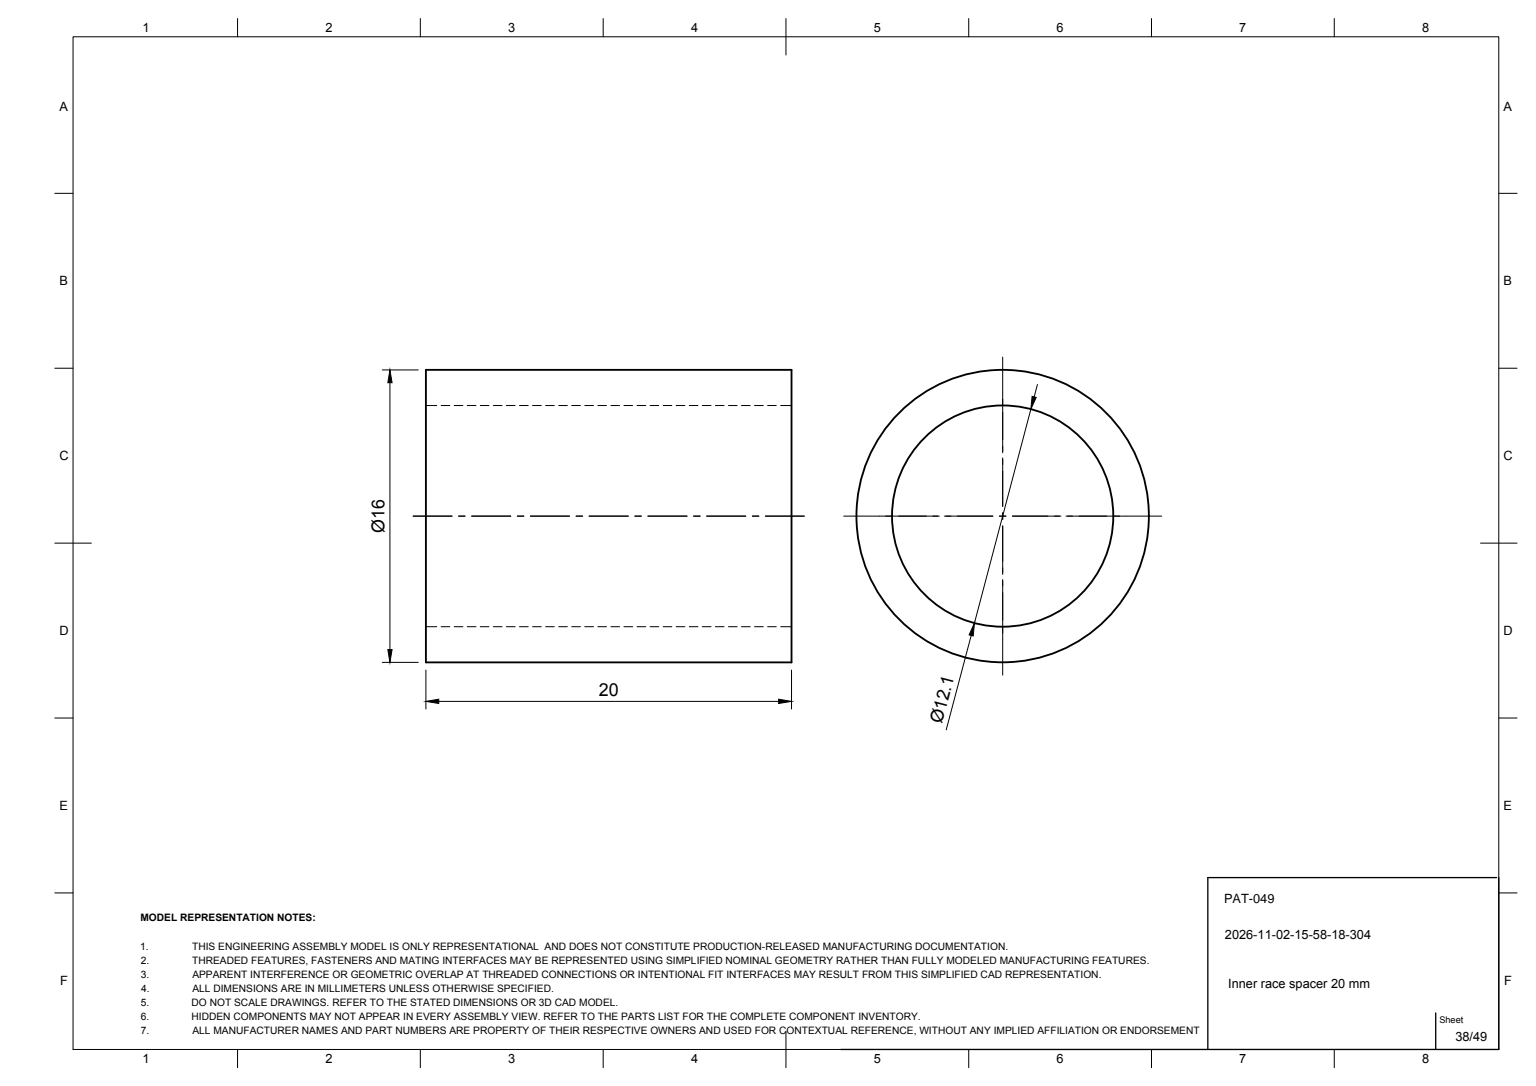
ISO-10303-21;
HEADER;
/* Generated by software containing ST-Developer
 * from STEP Tools, Inc. (www.steptools.com) 
 */

FILE_DESCRIPTION(
/* description */ ('Hand drill press frame (manual)'),
/* implementation_level */ '2;1');

FILE_NAME(
/* name */ 'Inner race spacer 20 mm.step',
/* time_stamp */ '2026-10-28T03:25:28-07:00',
/* author */ (''),
/* organization */ (''),
/* preprocessor_version */ 'ST-DEVELOPER v20.2',
/* originating_system */ 'Autodesk Translation Framework v15.17.0.0',
/* authorisation */ '');

FILE_SCHEMA (('AUTOMOTIVE_DESIGN { 1 0 10303 214 3 1 1 }'));
ENDSEC;

DATA;
#10=MECHANICAL_DESIGN_GEOMETRIC_PRESENTATION_REPRESENTATION('',(#656),#33299);
#559=SHAPE_REPRESENTATION_RELATIONSHIP('SRR','None',#33521,#604);
#604=ADVANCED_BREP_SHAPE_REPRESENTATION('',(#707),#33283);
#656=STYLED_ITEM('',(#33814),#707);
#707=MANIFOLD_SOLID_BREP('Body1',#12675);
#859=FACE_BOUND('',#2676,.T.);
#860=FACE_BOUND('',#2678,.T.);
#1252=PLANE('',#14040);
#1253=PLANE('',#14041);
#1845=FACE_OUTER_BOUND('',#2673,.T.);
#1846=FACE_OUTER_BOUND('',#2674,.T.);
#1847=FACE_OUTER_BOUND('',#2675,.T.);
#1848=FACE_OUTER_BOUND('',#2677,.T.);
#2673=EDGE_LOOP('',(#10931,#10932,#10933,#10934));
#2674=EDGE_LOOP('',(#10935,#10936,#10937,#10938));
#2675=EDGE_LOOP('',(#10939));
#2676=EDGE_LOOP('',(#10940));
#2677=EDGE_LOOP('',(#10941));
#2678=EDGE_LOOP('',(#10942));
#3808=LINE('',#21144,#4973);
#3809=LINE('',#21150,#4974);
#4973=VECTOR('',#16987,0.605);
#4974=VECTOR('',#16994,0.8);
#5507=CIRCLE('',#14035,0.605);
#5508=CIRCLE('',#14036,0.605);
#5509=CIRCLE('',#14038,0.8);
#5510=CIRCLE('',#14039,0.8);
#6457=VERTEX_POINT('',#21141);
#6458=VERTEX_POINT('',#21143);
#6459=VERTEX_POINT('',#21147);
#6460=VERTEX_POINT('',#21149);
#7994=EDGE_CURVE('',#6457,#6457,#5507,.T.);
#7995=EDGE_CURVE('',#6457,#6458,#3808,.T.);
#7996=EDGE_CURVE('',#6458,#6458,#5508,.T.);
#7997=EDGE_CURVE('',#6459,#6459,#5509,.T.);
#7998=EDGE_CURVE('',#6459,#6460,#3809,.T.);
#7999=EDGE_CURVE('',#6460,#6460,#5510,.T.);
#10931=ORIENTED_EDGE('',*,*,#7994,.F.);
#10932=ORIENTED_EDGE('',*,*,#7995,.T.);
#10933=ORIENTED_EDGE('',*,*,#7996,.T.);
#10934=ORIENTED_EDGE('',*,*,#7995,.F.);
#10935=ORIENTED_EDGE('',*,*,#7997,.F.);
#10936=ORIENTED_EDGE('',*,*,#7998,.T.);
#10937=ORIENTED_EDGE('',*,*,#7999,.T.);
#10938=ORIENTED_EDGE('',*,*,#7998,.F.);
#10939=ORIENTED_EDGE('',*,*,#7997,.T.);
#10940=ORIENTED_EDGE('',*,*,#7994,.T.);
#10941=ORIENTED_EDGE('',*,*,#7999,.F.);
#10942=ORIENTED_EDGE('',*,*,#7996,.F.);
#11900=CYLINDRICAL_SURFACE('',#14034,0.605);
#11901=CYLINDRICAL_SURFACE('',#14037,0.8);
#12454=ADVANCED_FACE('',(#1845),#11900,.F.);
#12455=ADVANCED_FACE('',(#1846),#11901,.T.);
#12456=ADVANCED_FACE('',(#1847,#859),#1252,.T.);
#12457=ADVANCED_FACE('',(#1848,#860),#1253,.F.);
#12675=CLOSED_SHELL('',(#12454,#12455,#12456,#12457));
#14033=AXIS2_PLACEMENT_3D('',#21139,#16981,#16982);
#14034=AXIS2_PLACEMENT_3D('',#21140,#16983,#16984);
#14035=AXIS2_PLACEMENT_3D('',#21142,#16985,#16986);
#14036=AXIS2_PLACEMENT_3D('',#21145,#16988,#16989);
#14037=AXIS2_PLACEMENT_3D('',#21146,#16990,#16991);
#14038=AXIS2_PLACEMENT_3D('',#21148,#16992,#16993);
#14039=AXIS2_PLACEMENT_3D('',#21151,#16995,#16996);
#14040=AXIS2_PLACEMENT_3D('',#21152,#16997,#16998);
#14041=AXIS2_PLACEMENT_3D('',#21153,#16999,#17000);
#16981=DIRECTION('axis',(0.,0.,1.));
#16982=DIRECTION('refdir',(1.,0.,0.));
#16983=DIRECTION('center_axis',(0.,1.,0.));
#16984=DIRECTION('ref_axis',(1.,0.,0.));
#16985=DIRECTION('center_axis',(0.,-1.,0.));
#16986=DIRECTION('ref_axis',(1.,0.,0.));
#16987=DIRECTION('',(0.,-1.,0.));
#16988=DIRECTION('center_axis',(0.,-1.,0.));
#16989=DIRECTION('ref_axis',(1.,0.,0.));
#16990=DIRECTION('center_axis',(0.,1.,0.));
#16991=DIRECTION('ref_axis',(1.,0.,0.));
#16992=DIRECTION('center_axis',(0.,1.,0.));
#16993=DIRECTION('ref_axis',(1.,0.,0.));
#16994=DIRECTION('',(0.,-1.,0.));
#16995=DIRECTION('center_axis',(0.,1.,0.));
#16996=DIRECTION('ref_axis',(1.,0.,0.));
#16997=DIRECTION('center_axis',(0.,1.,0.));
#16998=DIRECTION('ref_axis',(1.,0.,0.));
#16999=DIRECTION('center_axis',(0.,1.,0.));
#17000=DIRECTION('ref_axis',(1.,0.,0.));
#21139=CARTESIAN_POINT('',(0.,0.,0.));
#21140=CARTESIAN_POINT('Origin',(-3.25,-5.5,20.));
#21141=CARTESIAN_POINT('',(-3.855,-3.5,20.));
#21142=CARTESIAN_POINT('Origin',(-3.25,-3.5,20.));
#21143=CARTESIAN_POINT('',(-3.855,-5.5,20.));
#21144=CARTESIAN_POINT('',(-3.855,-5.5,20.));
#21145=CARTESIAN_POINT('Origin',(-3.25,-5.5,20.));
#21146=CARTESIAN_POINT('Origin',(-3.25,-5.5,20.));
#21147=CARTESIAN_POINT('',(-4.05,-3.5,20.));
#21148=CARTESIAN_POINT('Origin',(-3.25,-3.5,20.));
#21149=CARTESIAN_POINT('',(-4.05,-5.5,20.));
#21150=CARTESIAN_POINT('',(-4.05,-5.5,20.));
#21151=CARTESIAN_POINT('Origin',(-3.25,-5.5,20.));
#21152=CARTESIAN_POINT('Origin',(-3.25,-3.5,20.));
#21153=CARTESIAN_POINT('Origin',(-3.25,-5.5,20.));
#33231=UNCERTAINTY_MEASURE_WITH_UNIT(LENGTH_MEASURE(0.001),#33300,
'DISTANCE_ACCURACY_VALUE',
'Maximum model space distance between geometric entities at asserted c
onnectivities');
#33247=UNCERTAINTY_MEASURE_WITH_UNIT(LENGTH_MEASURE(0.001),#33300,
'DISTANCE_ACCURACY_VALUE',
'Maximum model space distance between geometric entities at asserted c
onnectivities');
#33283=(
GEOMETRIC_REPRESENTATION_CONTEXT(3)
GLOBAL_UNCERTAINTY_ASSIGNED_CONTEXT((#33231))
GLOBAL_UNIT_ASSIGNED_CONTEXT((#33300,#33302,#33303))
REPRESENTATION_CONTEXT('','3D')
);
#33299=(
GEOMETRIC_REPRESENTATION_CONTEXT(3)
GLOBAL_UNCERTAINTY_ASSIGNED_CONTEXT((#33247))
GLOBAL_UNIT_ASSIGNED_CONTEXT((#33300,#33302,#33303))
REPRESENTATION_CONTEXT('','3D')
);
#33300=(
LENGTH_UNIT()
NAMED_UNIT(*)
SI_UNIT(.CENTI.,.METRE.)
);
#33302=(
NAMED_UNIT(*)
PLANE_ANGLE_UNIT()
SI_UNIT($,.RADIAN.)
);
#33303=(
NAMED_UNIT(*)
SI_UNIT($,.STERADIAN.)
SOLID_ANGLE_UNIT()
);
#33339=SHAPE_DEFINITION_REPRESENTATION(#33401,#33521);
#33401=PRODUCT_DEFINITION_SHAPE('',$,#33573);
#33521=SHAPE_REPRESENTATION('',(#14033),#33283);
#33537=PRODUCT_DEFINITION_CONTEXT('part definition',#33692,'design');
#33573=PRODUCT_DEFINITION('Inner race spacer 20 mm',
'Inner race spacer 20 mm',#33624,#33537);
#33624=PRODUCT_DEFINITION_FORMATION('',$,#33729);
#33692=APPLICATION_CONTEXT(
'Core Data for Automotive Mechanical Design Process');
#33693=PRODUCT_CONTEXT('part definition',#33692,'mechanical');
#33729=PRODUCT('Inner race spacer 20 mm','Inner race spacer 20 mm',
'Inner race spacer 20 mm',(#33693));
#33808=COLOUR_RGB('Grey',0.48,0.52,0.57);
#33809=FILL_AREA_STYLE_COLOUR('',#33808);
#33810=FILL_AREA_STYLE('',(#33809));
#33811=SURFACE_STYLE_FILL_AREA(#33810);
#33812=SURFACE_SIDE_STYLE('',(#33811));
#33813=SURFACE_STYLE_USAGE(.BOTH.,#33812);
#33814=PRESENTATION_STYLE_ASSIGNMENT((#33813));
ENDSEC;
END-ISO-10303-21;
